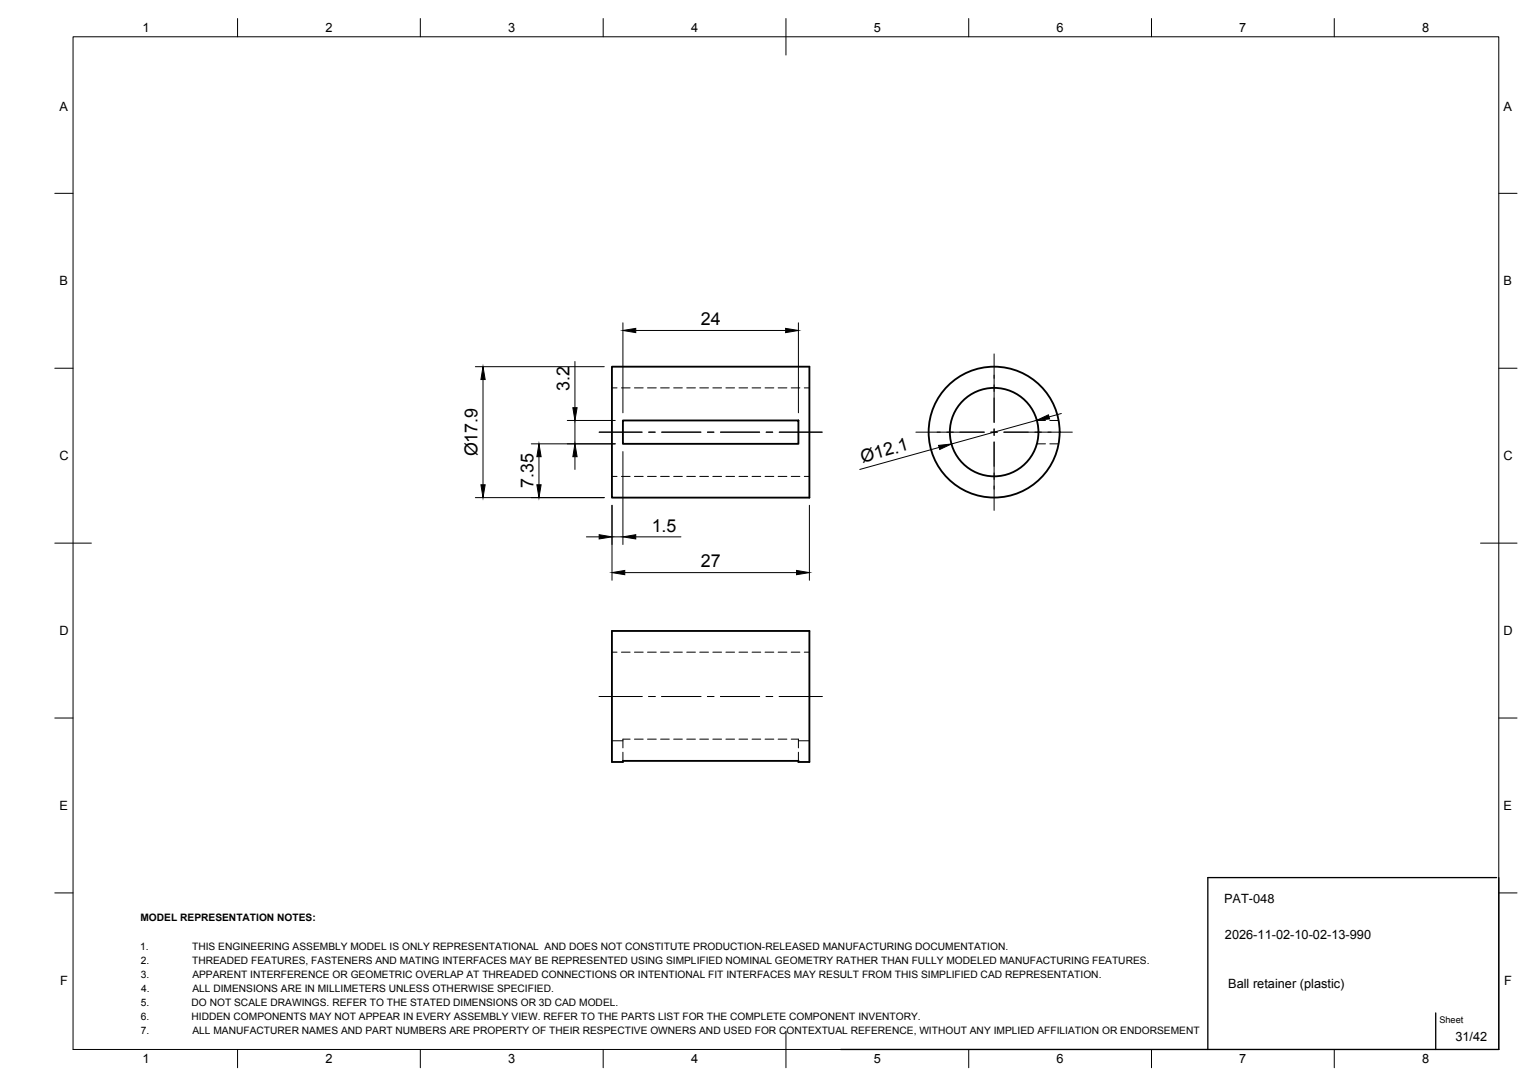
ISO-10303-21;
HEADER;
/* Generated by software containing ST-Developer
 * from STEP Tools, Inc. (www.steptools.com) 
 */

FILE_DESCRIPTION(
/* description */ ('Guided pneumatic stop gate'),
/* implementation_level */ '2;1');

FILE_NAME(
/* name */ 'Ball retainer (plastic).step',
/* time_stamp */ '2026-10-27T21:43:45-07:00',
/* author */ (''),
/* organization */ (''),
/* preprocessor_version */ 'ST-DEVELOPER v20.2',
/* originating_system */ 'Autodesk Translation Framework v15.17.0.0',
/* authorisation */ '');

FILE_SCHEMA (('AUTOMOTIVE_DESIGN { 1 0 10303 214 3 1 1 }'));
ENDSEC;

DATA;
#10=MECHANICAL_DESIGN_GEOMETRIC_PRESENTATION_REPRESENTATION('',(#560),#14392);
#476=SHAPE_REPRESENTATION_RELATIONSHIP('SRR','None',#14612,#518);
#518=ADVANCED_BREP_SHAPE_REPRESENTATION('',(#601),#14374);
#560=STYLED_ITEM('',(#14884),#601);
#601=MANIFOLD_SOLID_BREP('Body1',#7901);
#784=FACE_BOUND('',#2082,.T.);
#785=FACE_BOUND('',#2084,.T.);
#786=FACE_BOUND('',#2086,.T.);
#787=FACE_BOUND('',#2088,.T.);
#1014=PLANE('',#9014);
#1015=PLANE('',#9017);
#1016=PLANE('',#9018);
#1017=PLANE('',#9021);
#1018=PLANE('',#9022);
#1019=PLANE('',#9027);
#1433=FACE_OUTER_BOUND('',#2077,.T.);
#1434=FACE_OUTER_BOUND('',#2078,.T.);
#1435=FACE_OUTER_BOUND('',#2079,.T.);
#1436=FACE_OUTER_BOUND('',#2080,.T.);
#1437=FACE_OUTER_BOUND('',#2081,.T.);
#1438=FACE_OUTER_BOUND('',#2083,.T.);
#1439=FACE_OUTER_BOUND('',#2085,.T.);
#1440=FACE_OUTER_BOUND('',#2087,.T.);
#2077=EDGE_LOOP('',(#6606,#6607,#6608,#6609));
#2078=EDGE_LOOP('',(#6610,#6611,#6612,#6613));
#2079=EDGE_LOOP('',(#6614,#6615,#6616,#6617));
#2080=EDGE_LOOP('',(#6618,#6619,#6620,#6621));
#2081=EDGE_LOOP('',(#6622));
#2082=EDGE_LOOP('',(#6623));
#2083=EDGE_LOOP('',(#6624,#6625,#6626,#6627));
#2084=EDGE_LOOP('',(#6628,#6629,#6630,#6631));
#2085=EDGE_LOOP('',(#6632));
#2086=EDGE_LOOP('',(#6633));
#2087=EDGE_LOOP('',(#6634,#6635,#6636,#6637));
#2088=EDGE_LOOP('',(#6638,#6639,#6640,#6641));
#2628=LINE('',#13356,#3173);
#2629=LINE('',#13359,#3174);
#2630=LINE('',#13362,#3175);
#2631=LINE('',#13364,#3176);
#2632=LINE('',#13365,#3177);
#2633=LINE('',#13371,#3178);
#2634=LINE('',#13373,#3179);
#2635=LINE('',#13374,#3180);
#2636=LINE('',#13383,#3181);
#2637=LINE('',#13388,#3182);
#3173=VECTOR('',#10995,1.);
#3174=VECTOR('',#10998,1.);
#3175=VECTOR('',#11001,1.);
#3176=VECTOR('',#11002,1.);
#3177=VECTOR('',#11003,1.);
#3178=VECTOR('',#11010,1.);
#3179=VECTOR('',#11013,1.);
#3180=VECTOR('',#11014,1.);
#3181=VECTOR('',#11025,0.895);
#3182=VECTOR('',#11032,0.605);
#3637=CIRCLE('',#9015,0.895);
#3638=CIRCLE('',#9016,0.605);
#3639=CIRCLE('',#9019,0.895);
#3640=CIRCLE('',#9020,0.605);
#3641=CIRCLE('',#9023,0.895);
#3642=CIRCLE('',#9024,0.605);
#3643=CIRCLE('',#9026,0.895);
#3644=CIRCLE('',#9028,0.605);
#4152=VERTEX_POINT('',#13352);
#4153=VERTEX_POINT('',#13353);
#4154=VERTEX_POINT('',#13355);
#4155=VERTEX_POINT('',#13357);
#4156=VERTEX_POINT('',#13361);
#4157=VERTEX_POINT('',#13363);
#4158=VERTEX_POINT('',#13367);
#4159=VERTEX_POINT('',#13369);
#4160=VERTEX_POINT('',#13376);
#4161=VERTEX_POINT('',#13378);
#4162=VERTEX_POINT('',#13381);
#4163=VERTEX_POINT('',#13385);
#5001=EDGE_CURVE('',#4152,#4153,#3637,.T.);
#5002=EDGE_CURVE('',#4154,#4152,#2628,.T.);
#5003=EDGE_CURVE('',#4155,#4154,#3638,.T.);
#5004=EDGE_CURVE('',#4153,#4155,#2629,.T.);
#5005=EDGE_CURVE('',#4153,#4156,#2630,.T.);
#5006=EDGE_CURVE('',#4157,#4155,#2631,.T.);
#5007=EDGE_CURVE('',#4157,#4156,#2632,.T.);
#5008=EDGE_CURVE('',#4156,#4158,#3639,.T.);
#5009=EDGE_CURVE('',#4159,#4157,#3640,.T.);
#5010=EDGE_CURVE('',#4158,#4159,#2633,.T.);
#5011=EDGE_CURVE('',#4158,#4152,#2634,.T.);
#5012=EDGE_CURVE('',#4154,#4159,#2635,.T.);
#5013=EDGE_CURVE('',#4160,#4160,#3641,.T.);
#5014=EDGE_CURVE('',#4161,#4161,#3642,.T.);
#5015=EDGE_CURVE('',#4162,#4162,#3643,.T.);
#5016=EDGE_CURVE('',#4162,#4160,#2636,.T.);
#5017=EDGE_CURVE('',#4163,#4163,#3644,.T.);
#5018=EDGE_CURVE('',#4163,#4161,#2637,.T.);
#6606=ORIENTED_EDGE('',*,*,#5001,.F.);
#6607=ORIENTED_EDGE('',*,*,#5002,.F.);
#6608=ORIENTED_EDGE('',*,*,#5003,.F.);
#6609=ORIENTED_EDGE('',*,*,#5004,.F.);
#6610=ORIENTED_EDGE('',*,*,#5005,.F.);
#6611=ORIENTED_EDGE('',*,*,#5004,.T.);
#6612=ORIENTED_EDGE('',*,*,#5006,.F.);
#6613=ORIENTED_EDGE('',*,*,#5007,.T.);
#6614=ORIENTED_EDGE('',*,*,#5008,.F.);
#6615=ORIENTED_EDGE('',*,*,#5007,.F.);
#6616=ORIENTED_EDGE('',*,*,#5009,.F.);
#6617=ORIENTED_EDGE('',*,*,#5010,.F.);
#6618=ORIENTED_EDGE('',*,*,#5011,.F.);
#6619=ORIENTED_EDGE('',*,*,#5010,.T.);
#6620=ORIENTED_EDGE('',*,*,#5012,.F.);
#6621=ORIENTED_EDGE('',*,*,#5002,.T.);
#6622=ORIENTED_EDGE('',*,*,#5013,.F.);
#6623=ORIENTED_EDGE('',*,*,#5014,.T.);
#6624=ORIENTED_EDGE('',*,*,#5015,.F.);
#6625=ORIENTED_EDGE('',*,*,#5016,.T.);
#6626=ORIENTED_EDGE('',*,*,#5013,.T.);
#6627=ORIENTED_EDGE('',*,*,#5016,.F.);
#6628=ORIENTED_EDGE('',*,*,#5008,.T.);
#6629=ORIENTED_EDGE('',*,*,#5011,.T.);
#6630=ORIENTED_EDGE('',*,*,#5001,.T.);
#6631=ORIENTED_EDGE('',*,*,#5005,.T.);
#6632=ORIENTED_EDGE('',*,*,#5015,.T.);
#6633=ORIENTED_EDGE('',*,*,#5017,.F.);
#6634=ORIENTED_EDGE('',*,*,#5017,.T.);
#6635=ORIENTED_EDGE('',*,*,#5018,.T.);
#6636=ORIENTED_EDGE('',*,*,#5014,.F.);
#6637=ORIENTED_EDGE('',*,*,#5018,.F.);
#6638=ORIENTED_EDGE('',*,*,#5009,.T.);
#6639=ORIENTED_EDGE('',*,*,#5006,.T.);
#6640=ORIENTED_EDGE('',*,*,#5003,.T.);
#6641=ORIENTED_EDGE('',*,*,#5012,.T.);
#7363=CYLINDRICAL_SURFACE('',#9025,0.895);
#7364=CYLINDRICAL_SURFACE('',#9029,0.605);
#7715=ADVANCED_FACE('',(#1433),#1014,.F.);
#7716=ADVANCED_FACE('',(#1434),#1015,.F.);
#7717=ADVANCED_FACE('',(#1435),#1016,.F.);
#7718=ADVANCED_FACE('',(#1436),#1017,.F.);
#7719=ADVANCED_FACE('',(#1437,#784),#1018,.T.);
#7720=ADVANCED_FACE('',(#1438,#785),#7363,.T.);
#7721=ADVANCED_FACE('',(#1439,#786),#1019,.T.);
#7722=ADVANCED_FACE('',(#1440,#787),#7364,.F.);
#7901=CLOSED_SHELL('',(#7715,#7716,#7717,#7718,#7719,#7720,#7721,#7722));
#9013=AXIS2_PLACEMENT_3D('',#13350,#10989,#10990);
#9014=AXIS2_PLACEMENT_3D('',#13351,#10991,#10992);
#9015=AXIS2_PLACEMENT_3D('',#13354,#10993,#10994);
#9016=AXIS2_PLACEMENT_3D('',#13358,#10996,#10997);
#9017=AXIS2_PLACEMENT_3D('',#13360,#10999,#11000);
#9018=AXIS2_PLACEMENT_3D('',#13366,#11004,#11005);
#9019=AXIS2_PLACEMENT_3D('',#13368,#11006,#11007);
#9020=AXIS2_PLACEMENT_3D('',#13370,#11008,#11009);
#9021=AXIS2_PLACEMENT_3D('',#13372,#11011,#11012);
#9022=AXIS2_PLACEMENT_3D('',#13375,#11015,#11016);
#9023=AXIS2_PLACEMENT_3D('',#13377,#11017,#11018);
#9024=AXIS2_PLACEMENT_3D('',#13379,#11019,#11020);
#9025=AXIS2_PLACEMENT_3D('',#13380,#11021,#11022);
#9026=AXIS2_PLACEMENT_3D('',#13382,#11023,#11024);
#9027=AXIS2_PLACEMENT_3D('',#13384,#11026,#11027);
#9028=AXIS2_PLACEMENT_3D('',#13386,#11028,#11029);
#9029=AXIS2_PLACEMENT_3D('',#13387,#11030,#11031);
#10989=DIRECTION('axis',(0.,0.,1.));
#10990=DIRECTION('refdir',(1.,0.,0.));
#10991=DIRECTION('center_axis',(0.,1.,0.));
#10992=DIRECTION('ref_axis',(0.,0.,1.));
#10993=DIRECTION('center_axis',(0.,1.,0.));
#10994=DIRECTION('ref_axis',(1.,0.,0.));
#10995=DIRECTION('',(1.,0.,0.));
#10996=DIRECTION('center_axis',(0.,-1.,0.));
#10997=DIRECTION('ref_axis',(1.,0.,0.));
#10998=DIRECTION('',(-1.,0.,0.));
#10999=DIRECTION('center_axis',(0.,0.,-1.));
#11000=DIRECTION('ref_axis',(-1.,0.,0.));
#11001=DIRECTION('',(0.,-1.,0.));
#11002=DIRECTION('',(0.,1.,0.));
#11003=DIRECTION('',(1.,0.,0.));
#11004=DIRECTION('center_axis',(0.,-1.,0.));
#11005=DIRECTION('ref_axis',(0.,0.,-1.));
#11006=DIRECTION('center_axis',(0.,-1.,0.));
#11007=DIRECTION('ref_axis',(1.,0.,0.));
#11008=DIRECTION('center_axis',(0.,1.,0.));
#11009=DIRECTION('ref_axis',(1.,0.,0.));
#11010=DIRECTION('',(-1.,0.,0.));
#11011=DIRECTION('center_axis',(0.,0.,1.));
#11012=DIRECTION('ref_axis',(1.,0.,0.));
#11013=DIRECTION('',(0.,1.,0.));
#11014=DIRECTION('',(0.,-1.,0.));
#11015=DIRECTION('center_axis',(0.,1.,0.));
#11016=DIRECTION('ref_axis',(0.,0.,1.));
#11017=DIRECTION('center_axis',(0.,-1.,0.));
#11018=DIRECTION('ref_axis',(1.,0.,0.));
#11019=DIRECTION('center_axis',(0.,-1.,0.));
#11020=DIRECTION('ref_axis',(1.,0.,0.));
#11021=DIRECTION('center_axis',(0.,-1.,0.));
#11022=DIRECTION('ref_axis',(1.,0.,0.));
#11023=DIRECTION('center_axis',(0.,-1.,0.));
#11024=DIRECTION('ref_axis',(1.,0.,0.));
#11025=DIRECTION('',(0.,1.,0.));
#11026=DIRECTION('center_axis',(0.,-1.,0.));
#11027=DIRECTION('ref_axis',(0.,0.,-1.));
#11028=DIRECTION('center_axis',(0.,-1.,0.));
#11029=DIRECTION('ref_axis',(1.,0.,0.));
#11030=DIRECTION('center_axis',(0.,-1.,0.));
#11031=DIRECTION('ref_axis',(1.,0.,0.));
#11032=DIRECTION('',(0.,1.,0.));
#13350=CARTESIAN_POINT('',(0.,0.,0.));
#13351=CARTESIAN_POINT('Origin',(0.75,1.2,0.));
#13352=CARTESIAN_POINT('',(0.880582193778639,1.2,0.16));
#13353=CARTESIAN_POINT('',(0.880582193778639,1.2,-0.16));
#13354=CARTESIAN_POINT('Origin',(0.,1.2,0.));
#13355=CARTESIAN_POINT('',(0.583459510163302,1.2,0.16));
#13356=CARTESIAN_POINT('',(0.57,1.2,0.16));
#13357=CARTESIAN_POINT('',(0.583459510163302,1.2,-0.16));
#13358=CARTESIAN_POINT('Origin',(0.,1.2,0.));
#13359=CARTESIAN_POINT('',(0.93,1.2,-0.16));
#13360=CARTESIAN_POINT('Origin',(0.93,0.,-0.16));
#13361=CARTESIAN_POINT('',(0.880582193778639,-1.2,-0.16));
#13362=CARTESIAN_POINT('',(0.880582193778639,0.,-0.16));
#13363=CARTESIAN_POINT('',(0.583459510163302,-1.2,-0.16));
#13364=CARTESIAN_POINT('',(0.583459510163302,0.,-0.16));
#13365=CARTESIAN_POINT('',(0.93,-1.2,-0.16));
#13366=CARTESIAN_POINT('Origin',(0.75,-1.2,0.));
#13367=CARTESIAN_POINT('',(0.880582193778639,-1.2,0.16));
#13368=CARTESIAN_POINT('Origin',(0.,-1.2,0.));
#13369=CARTESIAN_POINT('',(0.583459510163302,-1.2,0.16));
#13370=CARTESIAN_POINT('Origin',(0.,-1.2,0.));
#13371=CARTESIAN_POINT('',(0.57,-1.2,0.16));
#13372=CARTESIAN_POINT('Origin',(0.57,0.,0.16));
#13373=CARTESIAN_POINT('',(0.880582193778639,0.,0.16));
#13374=CARTESIAN_POINT('',(0.583459510163302,0.,0.16));
#13375=CARTESIAN_POINT('Origin',(0.895,1.35,0.));
#13376=CARTESIAN_POINT('',(-0.895,1.35,-1.09605888523688E-16));
#13377=CARTESIAN_POINT('Origin',(0.,1.35,0.));
#13378=CARTESIAN_POINT('',(-0.605,1.35,-7.40911313484149E-17));
#13379=CARTESIAN_POINT('Origin',(0.,1.35,0.));
#13380=CARTESIAN_POINT('Origin',(0.,0.,0.));
#13381=CARTESIAN_POINT('',(-0.895,-1.35,-1.09605888523688E-16));
#13382=CARTESIAN_POINT('Origin',(0.,-1.35,0.));
#13383=CARTESIAN_POINT('',(-0.895,0.,-1.09605888523688E-16));
#13384=CARTESIAN_POINT('Origin',(0.605,-1.35,0.));
#13385=CARTESIAN_POINT('',(-0.605,-1.35,-7.40911313484149E-17));
#13386=CARTESIAN_POINT('Origin',(0.,-1.35,0.));
#13387=CARTESIAN_POINT('Origin',(0.,0.,0.));
#13388=CARTESIAN_POINT('',(-0.605,0.,-7.40911313484149E-17));
#14326=UNCERTAINTY_MEASURE_WITH_UNIT(LENGTH_MEASURE(0.001),#14393,
'DISTANCE_ACCURACY_VALUE',
'Maximum model space distance between geometric entities at asserted c
onnectivities');
#14344=UNCERTAINTY_MEASURE_WITH_UNIT(LENGTH_MEASURE(0.001),#14393,
'DISTANCE_ACCURACY_VALUE',
'Maximum model space distance between geometric entities at asserted c
onnectivities');
#14374=(
GEOMETRIC_REPRESENTATION_CONTEXT(3)
GLOBAL_UNCERTAINTY_ASSIGNED_CONTEXT((#14326))
GLOBAL_UNIT_ASSIGNED_CONTEXT((#14393,#14395,#14396))
REPRESENTATION_CONTEXT('','3D')
);
#14392=(
GEOMETRIC_REPRESENTATION_CONTEXT(3)
GLOBAL_UNCERTAINTY_ASSIGNED_CONTEXT((#14344))
GLOBAL_UNIT_ASSIGNED_CONTEXT((#14393,#14395,#14396))
REPRESENTATION_CONTEXT('','3D')
);
#14393=(
LENGTH_UNIT()
NAMED_UNIT(*)
SI_UNIT(.CENTI.,.METRE.)
);
#14395=(
NAMED_UNIT(*)
PLANE_ANGLE_UNIT()
SI_UNIT($,.RADIAN.)
);
#14396=(
NAMED_UNIT(*)
SI_UNIT($,.STERADIAN.)
SOLID_ANGLE_UNIT()
);
#14426=SHAPE_DEFINITION_REPRESENTATION(#14475,#14612);
#14475=PRODUCT_DEFINITION_SHAPE('',$,#14660);
#14612=SHAPE_REPRESENTATION('',(#9013),#14374);
#14630=PRODUCT_DEFINITION_CONTEXT('part definition',#14773,'design');
#14660=PRODUCT_DEFINITION('Ball retainer (plastic)',
'Ball retainer (plastic)',#14707,#14630);
#14707=PRODUCT_DEFINITION_FORMATION('',$,#14804);
#14773=APPLICATION_CONTEXT(
'Core Data for Automotive Mechanical Design Process');
#14774=PRODUCT_CONTEXT('part definition',#14773,'mechanical');
#14804=PRODUCT('Ball retainer (plastic)','Ball retainer (plastic)',
'Ball retainer (plastic)',(#14774));
#14878=COLOUR_RGB('Sky Blue',0.24,0.69,0.87);
#14879=FILL_AREA_STYLE_COLOUR('',#14878);
#14880=FILL_AREA_STYLE('',(#14879));
#14881=SURFACE_STYLE_FILL_AREA(#14880);
#14882=SURFACE_SIDE_STYLE('',(#14881));
#14883=SURFACE_STYLE_USAGE(.BOTH.,#14882);
#14884=PRESENTATION_STYLE_ASSIGNMENT((#14883));
ENDSEC;
END-ISO-10303-21;
